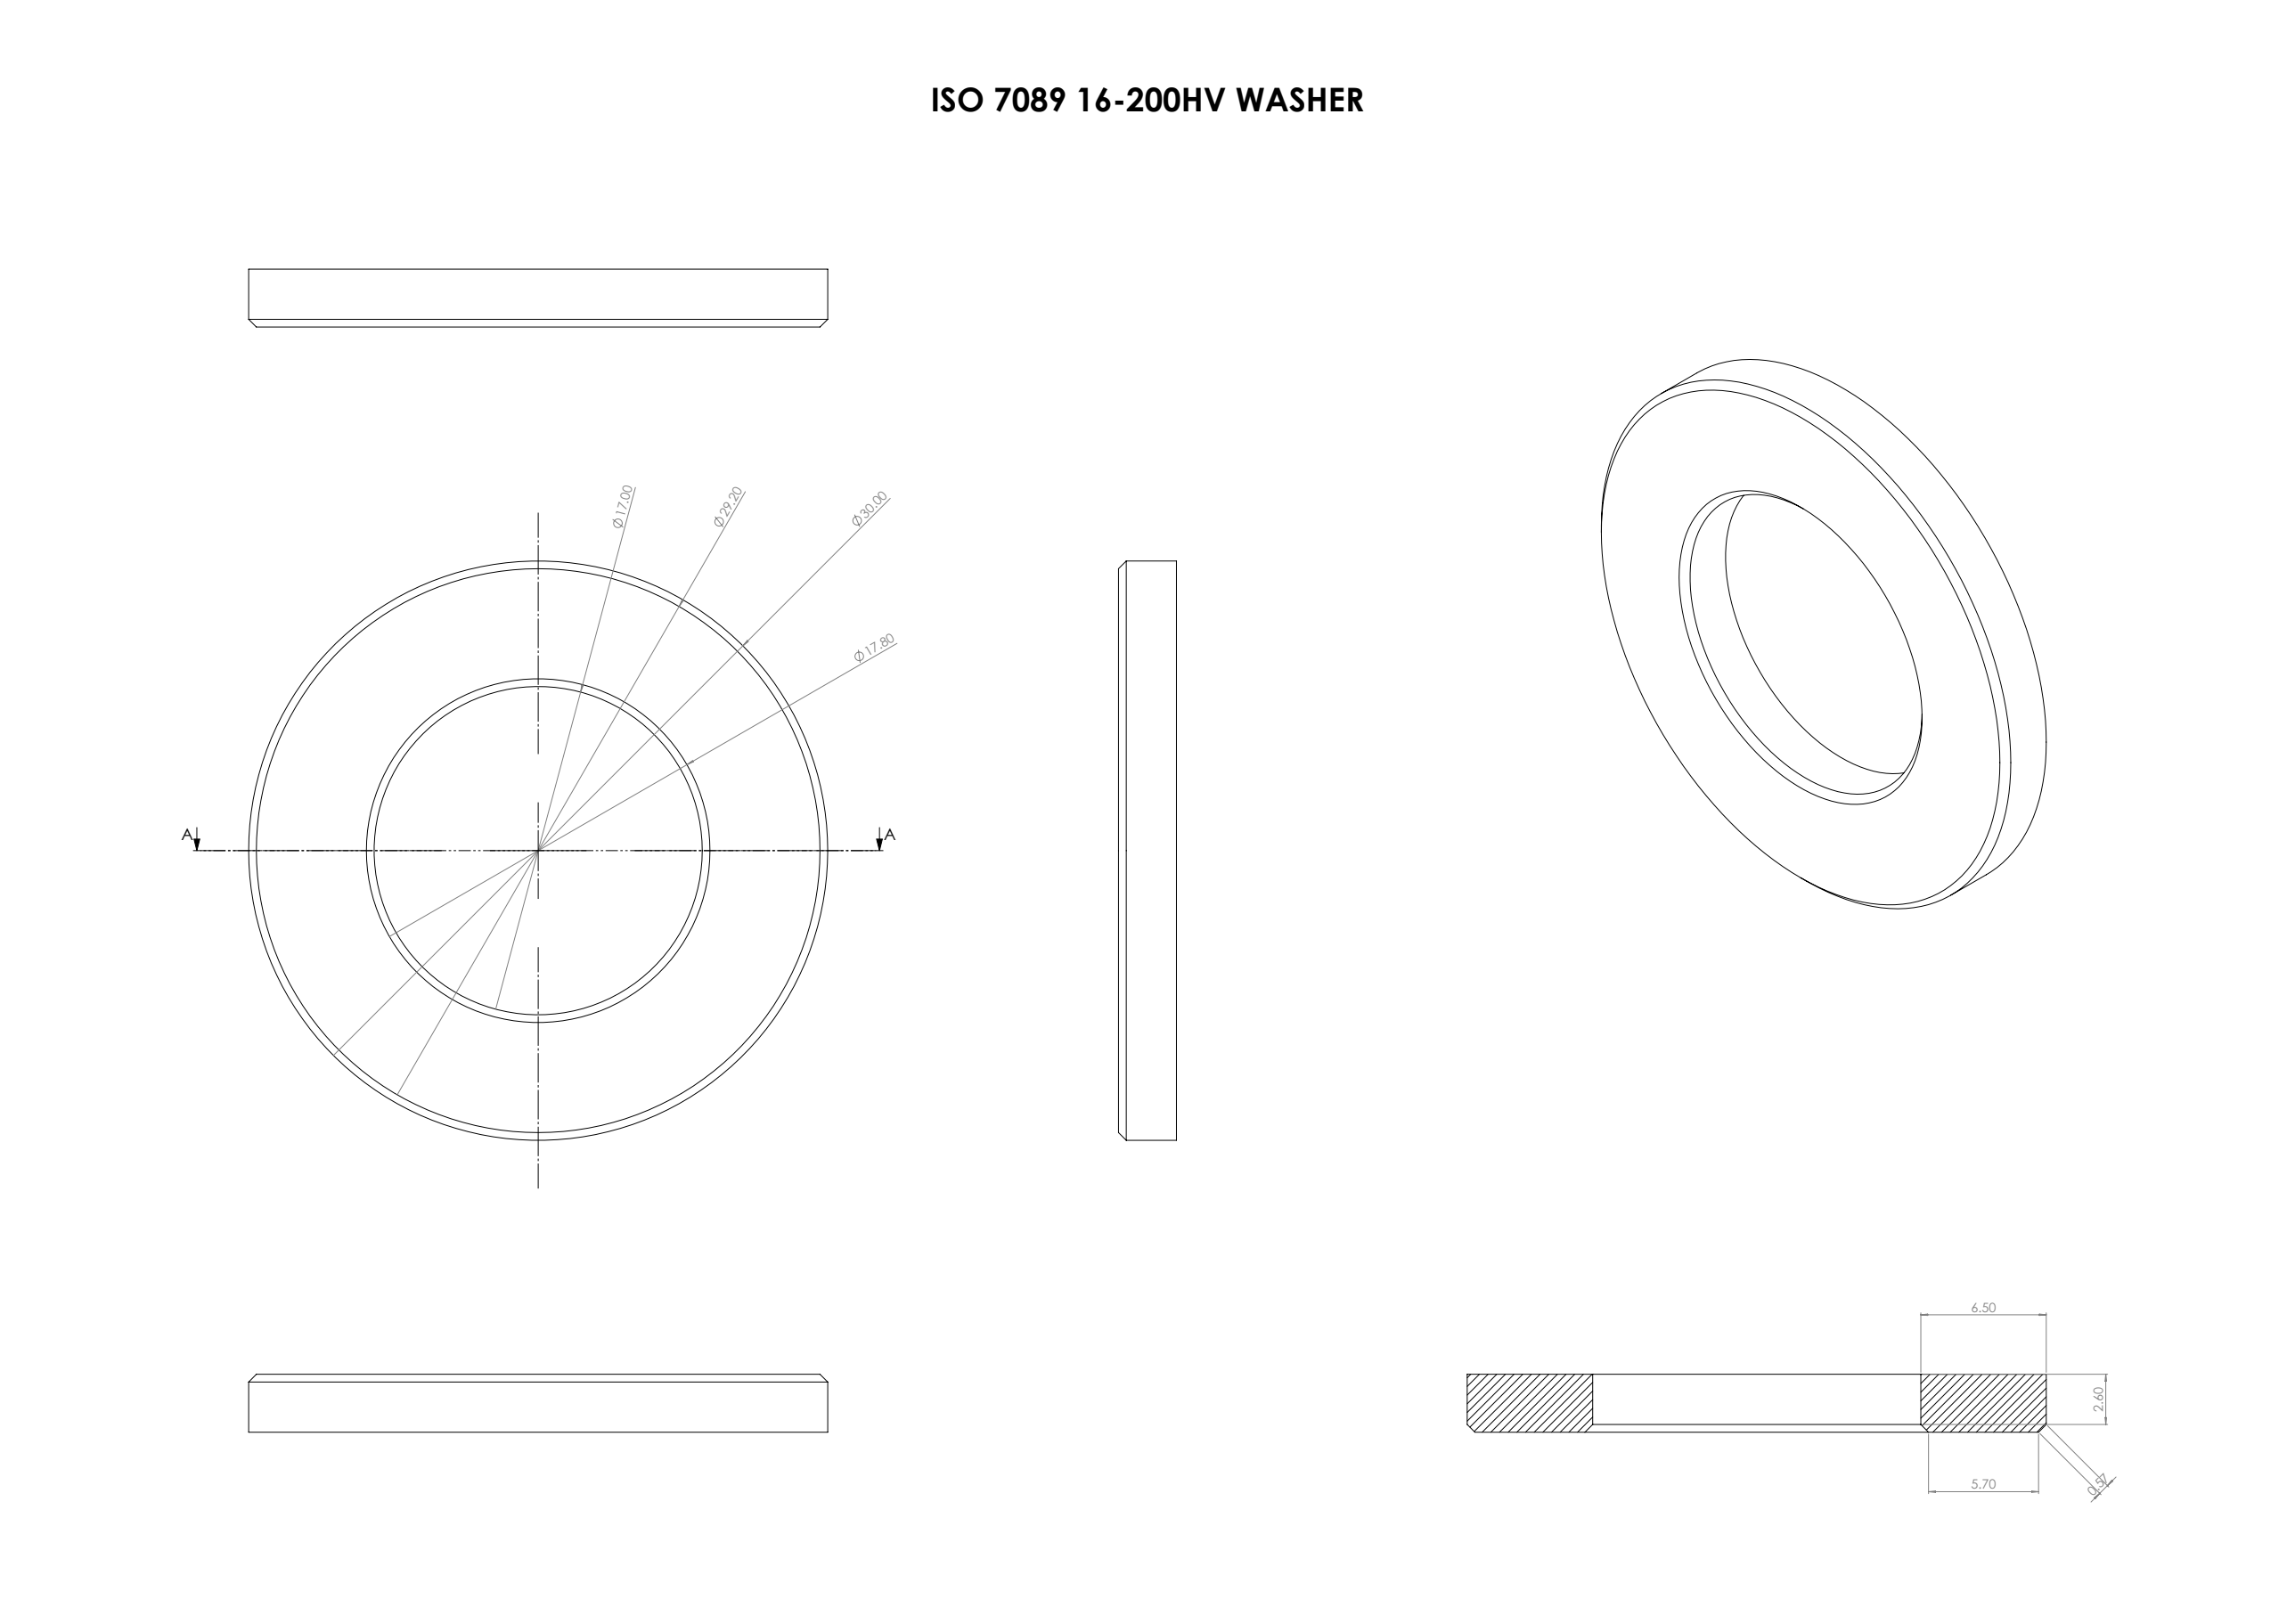
ISO-10303-21;
HEADER;
/* Generated by software containing ST-Developer
 * from STEP Tools, Inc. (www.steptools.com) 
 */

FILE_DESCRIPTION(
/* description */ (''),
/* implementation_level */ '2;1');

FILE_NAME(
/* name */ '19_ISO_7089_16-200HV_Washer.step',
/* time_stamp */ '2026-10-20T10:03:03-07:00',
/* author */ (''),
/* organization */ (''),
/* preprocessor_version */ 'ST-DEVELOPER v20.2',
/* originating_system */ 'Autodesk Translation Framework v15.15.0.0',
/* authorisation */ '');

FILE_SCHEMA (('AUTOMOTIVE_DESIGN { 1 0 10303 214 3 1 1 }'));
ENDSEC;

DATA;
#10=MECHANICAL_DESIGN_GEOMETRIC_PRESENTATION_REPRESENTATION('',(#541),#71492);
#398=SHAPE_REPRESENTATION_RELATIONSHIP('SRR','None',#71619,#417);
#417=ADVANCED_BREP_SHAPE_REPRESENTATION('',(#436),#71489);
#436=MANIFOLD_SOLID_BREP('Washer',#28475);
#541=STYLED_ITEM('',(#71894),#436);
#1831=CYLINDRICAL_SURFACE('',#30465,0.85);
#1832=CYLINDRICAL_SURFACE('',#30470,1.5);
#1986=FACE_BOUND('',#6084,.T.);
#1987=FACE_BOUND('',#6088,.T.);
#2569=CIRCLE('',#30466,0.85);
#2570=CIRCLE('',#30467,0.85);
#2571=CIRCLE('',#30469,1.5);
#2572=CIRCLE('',#30471,1.5);
#2573=CIRCLE('',#30473,1.46);
#2574=CIRCLE('',#30475,0.89);
#2899=CONICAL_SURFACE('',#30472,1.48,0.785398163397449);
#2900=CONICAL_SURFACE('',#30476,0.87,0.785398163397449);
#4390=FACE_OUTER_BOUND('',#6082,.T.);
#4391=FACE_OUTER_BOUND('',#6083,.T.);
#4392=FACE_OUTER_BOUND('',#6085,.T.);
#4393=FACE_OUTER_BOUND('',#6086,.T.);
#4394=FACE_OUTER_BOUND('',#6087,.T.);
#4395=FACE_OUTER_BOUND('',#6089,.T.);
#6082=EDGE_LOOP('',(#25367,#25368,#25369,#25370));
#6083=EDGE_LOOP('',(#25371));
#6084=EDGE_LOOP('',(#25372));
#6085=EDGE_LOOP('',(#25373,#25374,#25375,#25376));
#6086=EDGE_LOOP('',(#25377,#25378,#25379,#25380));
#6087=EDGE_LOOP('',(#25381));
#6088=EDGE_LOOP('',(#25382));
#6089=EDGE_LOOP('',(#25383,#25384,#25385,#25386));
#8600=LINE('',#70669,#11088);
#8601=LINE('',#70677,#11089);
#8602=LINE('',#70681,#11090);
#8603=LINE('',#70686,#11091);
#11088=VECTOR('',#36711,0.85);
#11089=VECTOR('',#36722,1.5);
#11090=VECTOR('',#36727,1.48);
#11091=VECTOR('',#36734,0.87);
#13637=VERTEX_POINT('',#70666);
#13638=VERTEX_POINT('',#70668);
#13639=VERTEX_POINT('',#70672);
#13640=VERTEX_POINT('',#70675);
#13641=VERTEX_POINT('',#70679);
#13642=VERTEX_POINT('',#70683);
#17567=EDGE_CURVE('',#13637,#13637,#2569,.T.);
#17568=EDGE_CURVE('',#13637,#13638,#8600,.T.);
#17569=EDGE_CURVE('',#13638,#13638,#2570,.T.);
#17570=EDGE_CURVE('',#13639,#13639,#2571,.T.);
#17571=EDGE_CURVE('',#13640,#13640,#2572,.T.);
#17572=EDGE_CURVE('',#13640,#13639,#8601,.T.);
#17573=EDGE_CURVE('',#13641,#13641,#2573,.T.);
#17574=EDGE_CURVE('',#13641,#13640,#8602,.T.);
#17575=EDGE_CURVE('',#13642,#13642,#2574,.T.);
#17576=EDGE_CURVE('',#13642,#13637,#8603,.T.);
#25367=ORIENTED_EDGE('',*,*,#17567,.T.);
#25368=ORIENTED_EDGE('',*,*,#17568,.T.);
#25369=ORIENTED_EDGE('',*,*,#17569,.F.);
#25370=ORIENTED_EDGE('',*,*,#17568,.F.);
#25371=ORIENTED_EDGE('',*,*,#17570,.F.);
#25372=ORIENTED_EDGE('',*,*,#17569,.T.);
#25373=ORIENTED_EDGE('',*,*,#17571,.F.);
#25374=ORIENTED_EDGE('',*,*,#17572,.T.);
#25375=ORIENTED_EDGE('',*,*,#17570,.T.);
#25376=ORIENTED_EDGE('',*,*,#17572,.F.);
#25377=ORIENTED_EDGE('',*,*,#17573,.F.);
#25378=ORIENTED_EDGE('',*,*,#17574,.T.);
#25379=ORIENTED_EDGE('',*,*,#17571,.T.);
#25380=ORIENTED_EDGE('',*,*,#17574,.F.);
#25381=ORIENTED_EDGE('',*,*,#17573,.T.);
#25382=ORIENTED_EDGE('',*,*,#17575,.F.);
#25383=ORIENTED_EDGE('',*,*,#17575,.T.);
#25384=ORIENTED_EDGE('',*,*,#17576,.T.);
#25385=ORIENTED_EDGE('',*,*,#17567,.F.);
#25386=ORIENTED_EDGE('',*,*,#17576,.F.);
#26833=PLANE('',#30468);
#26834=PLANE('',#30474);
#28298=ADVANCED_FACE('',(#4390),#1831,.F.);
#28299=ADVANCED_FACE('',(#4391,#1986),#26833,.T.);
#28300=ADVANCED_FACE('',(#4392),#1832,.T.);
#28301=ADVANCED_FACE('',(#4393),#2899,.T.);
#28302=ADVANCED_FACE('',(#4394,#1987),#26834,.T.);
#28303=ADVANCED_FACE('',(#4395),#2900,.F.);
#28475=CLOSED_SHELL('',(#28298,#28299,#28300,#28301,#28302,#28303));
#30464=AXIS2_PLACEMENT_3D('',#70664,#36705,#36706);
#30465=AXIS2_PLACEMENT_3D('',#70665,#36707,#36708);
#30466=AXIS2_PLACEMENT_3D('',#70667,#36709,#36710);
#30467=AXIS2_PLACEMENT_3D('',#70670,#36712,#36713);
#30468=AXIS2_PLACEMENT_3D('',#70671,#36714,#36715);
#30469=AXIS2_PLACEMENT_3D('',#70673,#36716,#36717);
#30470=AXIS2_PLACEMENT_3D('',#70674,#36718,#36719);
#30471=AXIS2_PLACEMENT_3D('',#70676,#36720,#36721);
#30472=AXIS2_PLACEMENT_3D('',#70678,#36723,#36724);
#30473=AXIS2_PLACEMENT_3D('',#70680,#36725,#36726);
#30474=AXIS2_PLACEMENT_3D('',#70682,#36728,#36729);
#30475=AXIS2_PLACEMENT_3D('',#70684,#36730,#36731);
#30476=AXIS2_PLACEMENT_3D('',#70685,#36732,#36733);
#36705=DIRECTION('axis',(0.,0.,1.));
#36706=DIRECTION('refdir',(1.,0.,0.));
#36707=DIRECTION('center_axis',(0.,0.,1.));
#36708=DIRECTION('ref_axis',(1.,0.,0.));
#36709=DIRECTION('center_axis',(0.,0.,1.));
#36710=DIRECTION('ref_axis',(1.,0.,0.));
#36711=DIRECTION('',(0.,0.,-1.));
#36712=DIRECTION('center_axis',(0.,0.,1.));
#36713=DIRECTION('ref_axis',(1.,0.,0.));
#36714=DIRECTION('center_axis',(0.,0.,-1.));
#36715=DIRECTION('ref_axis',(-1.,0.,0.));
#36716=DIRECTION('center_axis',(0.,0.,1.));
#36717=DIRECTION('ref_axis',(1.,0.,0.));
#36718=DIRECTION('center_axis',(0.,0.,1.));
#36719=DIRECTION('ref_axis',(1.,0.,0.));
#36720=DIRECTION('center_axis',(0.,0.,1.));
#36721=DIRECTION('ref_axis',(1.,0.,0.));
#36722=DIRECTION('',(0.,0.,-1.));
#36723=DIRECTION('center_axis',(0.,0.,-1.));
#36724=DIRECTION('ref_axis',(1.,0.,0.));
#36725=DIRECTION('center_axis',(0.,0.,1.));
#36726=DIRECTION('ref_axis',(1.,0.,0.));
#36727=DIRECTION('',(-0.707106781186548,-8.65956056235494E-17,-0.707106781186547));
#36728=DIRECTION('center_axis',(0.,0.,1.));
#36729=DIRECTION('ref_axis',(1.,0.,0.));
#36730=DIRECTION('center_axis',(0.,0.,1.));
#36731=DIRECTION('ref_axis',(1.,0.,0.));
#36732=DIRECTION('center_axis',(0.,0.,1.));
#36733=DIRECTION('ref_axis',(1.,0.,0.));
#36734=DIRECTION('',(0.707106781186548,8.65956056235494E-17,-0.707106781186547));
#70664=CARTESIAN_POINT('',(0.,0.,0.));
#70665=CARTESIAN_POINT('Origin',(0.,0.,0.13));
#70666=CARTESIAN_POINT('',(-0.85,-1.04094977927525E-16,0.26));
#70667=CARTESIAN_POINT('Origin',(0.,0.,0.26));
#70668=CARTESIAN_POINT('',(-0.85,-1.04094977927525E-16,0.));
#70669=CARTESIAN_POINT('',(-0.85,-1.04094977927525E-16,0.13));
#70670=CARTESIAN_POINT('Origin',(0.,0.,0.));
#70671=CARTESIAN_POINT('Origin',(1.5,0.,0.));
#70672=CARTESIAN_POINT('',(-1.5,-1.83697019872103E-16,0.));
#70673=CARTESIAN_POINT('Origin',(0.,0.,0.));
#70674=CARTESIAN_POINT('Origin',(0.,0.,0.13));
#70675=CARTESIAN_POINT('',(-1.5,-1.83697019872103E-16,0.26));
#70676=CARTESIAN_POINT('Origin',(0.,0.,0.26));
#70677=CARTESIAN_POINT('',(-1.5,-1.83697019872103E-16,0.13));
#70678=CARTESIAN_POINT('Origin',(0.,0.,0.28));
#70679=CARTESIAN_POINT('',(-1.46,-1.78798432675514E-16,0.3));
#70680=CARTESIAN_POINT('Origin',(0.,0.,0.3));
#70681=CARTESIAN_POINT('',(-1.48,-1.81247726273808E-16,0.28));
#70682=CARTESIAN_POINT('Origin',(0.89,0.,0.3));
#70683=CARTESIAN_POINT('',(-0.89,-1.08993565124114E-16,0.3));
#70684=CARTESIAN_POINT('Origin',(0.,0.,0.3));
#70685=CARTESIAN_POINT('Origin',(0.,0.,0.28));
#70686=CARTESIAN_POINT('',(-0.87,-1.0654427152582E-16,0.28));
#71468=UNCERTAINTY_MEASURE_WITH_UNIT(LENGTH_MEASURE(0.001),#71493,
'DISTANCE_ACCURACY_VALUE',
'Maximum model space distance between geometric entities at asserted c
onnectivities');
#71471=UNCERTAINTY_MEASURE_WITH_UNIT(LENGTH_MEASURE(0.001),#71493,
'DISTANCE_ACCURACY_VALUE',
'Maximum model space distance between geometric entities at asserted c
onnectivities');
#71489=(
GEOMETRIC_REPRESENTATION_CONTEXT(3)
GLOBAL_UNCERTAINTY_ASSIGNED_CONTEXT((#71468))
GLOBAL_UNIT_ASSIGNED_CONTEXT((#71493,#71495,#71496))
REPRESENTATION_CONTEXT('','3D')
);
#71492=(
GEOMETRIC_REPRESENTATION_CONTEXT(3)
GLOBAL_UNCERTAINTY_ASSIGNED_CONTEXT((#71471))
GLOBAL_UNIT_ASSIGNED_CONTEXT((#71493,#71495,#71496))
REPRESENTATION_CONTEXT('','3D')
);
#71493=(
LENGTH_UNIT()
NAMED_UNIT(*)
SI_UNIT(.CENTI.,.METRE.)
);
#71495=(
NAMED_UNIT(*)
PLANE_ANGLE_UNIT()
SI_UNIT($,.RADIAN.)
);
#71496=(
NAMED_UNIT(*)
SI_UNIT($,.STERADIAN.)
SOLID_ANGLE_UNIT()
);
#71514=SHAPE_DEFINITION_REPRESENTATION(#71534,#71619);
#71534=PRODUCT_DEFINITION_SHAPE('',$,#71640);
#71619=SHAPE_REPRESENTATION('',(#30464),#71489);
#71622=PRODUCT_DEFINITION_CONTEXT('part definition',#71684,'design');
#71640=PRODUCT_DEFINITION('2026-10-19-03-23-19-103',
'19_ISO_7089_16-200HV_Washer',#71660,#71622);
#71660=PRODUCT_DEFINITION_FORMATION('',$,#71703);
#71684=APPLICATION_CONTEXT(
'Core Data for Automotive Mechanical Design Process');
#71685=PRODUCT_CONTEXT('part definition',#71684,'mechanical');
#71703=PRODUCT('2026-10-19-03-23-19-103','19_ISO_7089_16-200HV_Washer',
$,(#71685));
#71888=COLOUR_RGB('Black',0.12,0.14,0.17);
#71889=FILL_AREA_STYLE_COLOUR('',#71888);
#71890=FILL_AREA_STYLE('',(#71889));
#71891=SURFACE_STYLE_FILL_AREA(#71890);
#71892=SURFACE_SIDE_STYLE('',(#71891));
#71893=SURFACE_STYLE_USAGE(.BOTH.,#71892);
#71894=PRESENTATION_STYLE_ASSIGNMENT((#71893));
ENDSEC;
END-ISO-10303-21;
